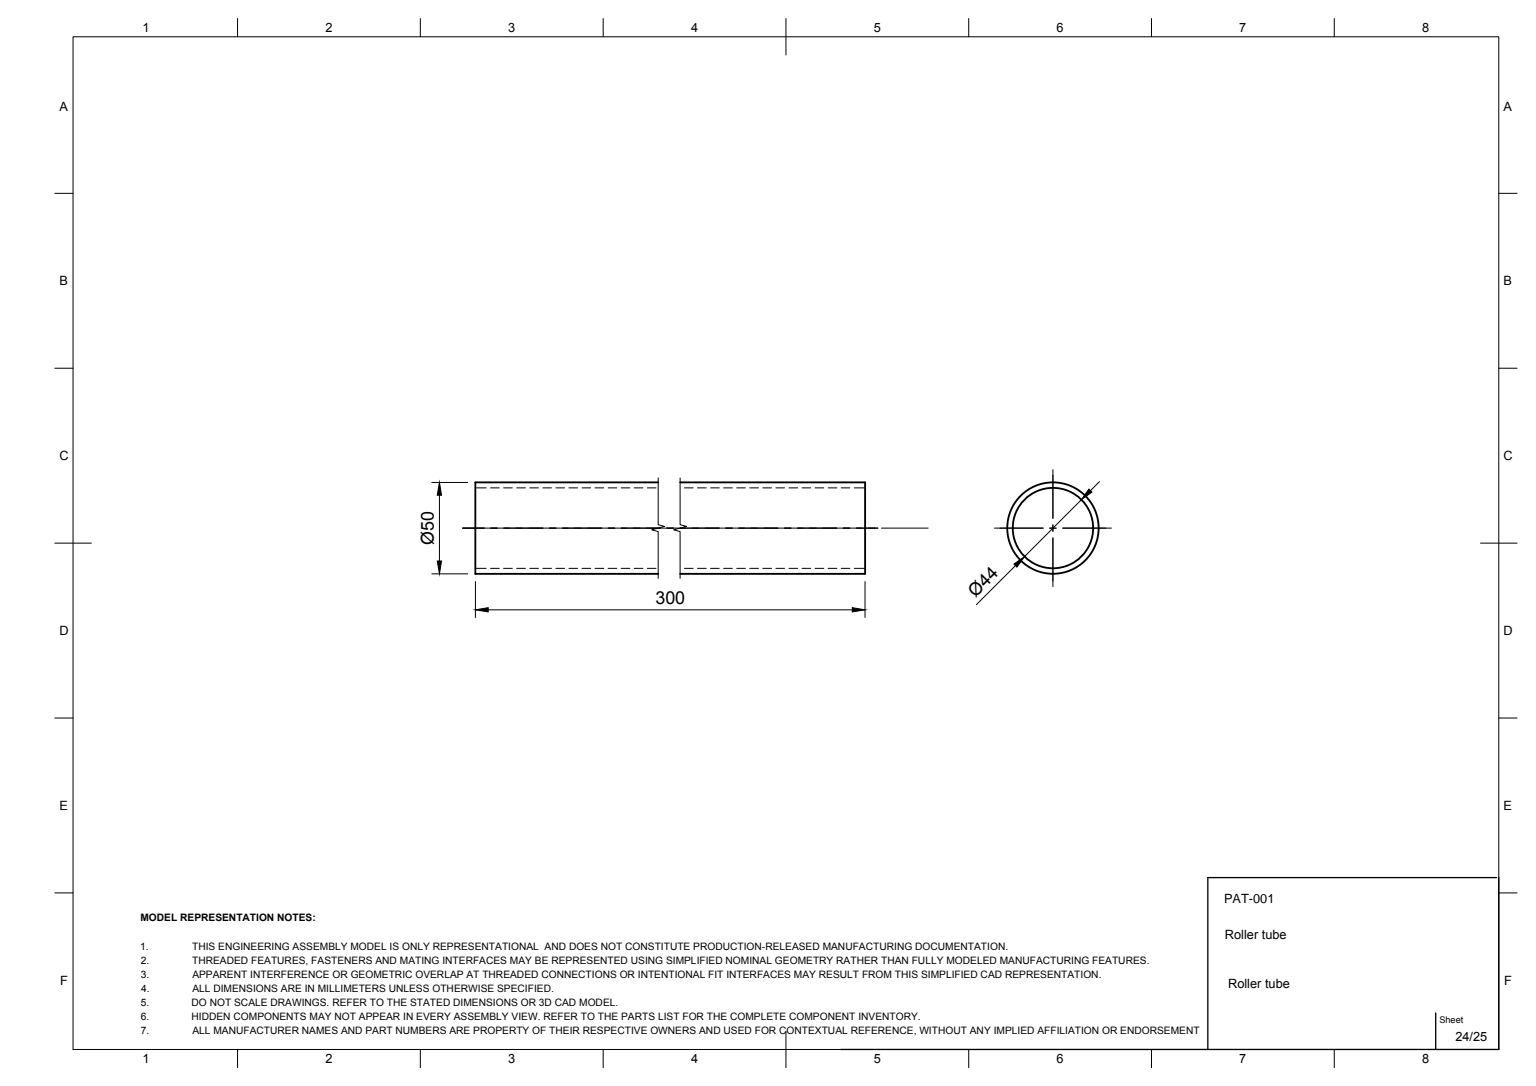
ISO-10303-21;
HEADER;
/* Generated by software containing ST-Developer
 * from STEP Tools, Inc. (www.steptools.com) 
 */

FILE_DESCRIPTION(
/* description */ ('PAT-001'),
/* implementation_level */ '2;1');

FILE_NAME(
/* name */ 'Roller tube.step',
/* time_stamp */ '2026-10-29T17:07:15-07:00',
/* author */ (''),
/* organization */ (''),
/* preprocessor_version */ 'ST-DEVELOPER v20.2',
/* originating_system */ 'Autodesk Translation Framework v15.17.0.0',
/* authorisation */ '');

FILE_SCHEMA (('AUTOMOTIVE_DESIGN { 1 0 10303 214 3 1 1 }'));
ENDSEC;

DATA;
#10=MECHANICAL_DESIGN_GEOMETRIC_PRESENTATION_REPRESENTATION('',(#403),#9622);
#345=SHAPE_REPRESENTATION_RELATIONSHIP('SRR','None',#9770,#370);
#370=ADVANCED_BREP_SHAPE_REPRESENTATION('',(#435),#9619);
#403=STYLED_ITEM('',(#9948),#435);
#435=MANIFOLD_SOLID_BREP('Body1',#5229);
#515=FACE_BOUND('',#1359,.T.);
#516=FACE_BOUND('',#1361,.T.);
#700=PLANE('',#6004);
#701=PLANE('',#6005);
#982=FACE_OUTER_BOUND('',#1356,.T.);
#983=FACE_OUTER_BOUND('',#1357,.T.);
#984=FACE_OUTER_BOUND('',#1358,.T.);
#985=FACE_OUTER_BOUND('',#1360,.T.);
#1356=EDGE_LOOP('',(#4715,#4716,#4717,#4718));
#1357=EDGE_LOOP('',(#4719,#4720,#4721,#4722));
#1358=EDGE_LOOP('',(#4723));
#1359=EDGE_LOOP('',(#4724));
#1360=EDGE_LOOP('',(#4725));
#1361=EDGE_LOOP('',(#4726));
#1771=LINE('',#9390,#2176);
#1772=LINE('',#9396,#2177);
#2176=VECTOR('',#7462,2.2);
#2177=VECTOR('',#7469,2.5);
#2396=CIRCLE('',#5999,2.2);
#2397=CIRCLE('',#6000,2.2);
#2398=CIRCLE('',#6002,2.5);
#2399=CIRCLE('',#6003,2.5);
#2826=VERTEX_POINT('',#9387);
#2827=VERTEX_POINT('',#9389);
#2828=VERTEX_POINT('',#9393);
#2829=VERTEX_POINT('',#9395);
#3461=EDGE_CURVE('',#2826,#2826,#2396,.T.);
#3462=EDGE_CURVE('',#2826,#2827,#1771,.T.);
#3463=EDGE_CURVE('',#2827,#2827,#2397,.T.);
#3464=EDGE_CURVE('',#2828,#2828,#2398,.T.);
#3465=EDGE_CURVE('',#2828,#2829,#1772,.T.);
#3466=EDGE_CURVE('',#2829,#2829,#2399,.T.);
#4715=ORIENTED_EDGE('',*,*,#3461,.F.);
#4716=ORIENTED_EDGE('',*,*,#3462,.T.);
#4717=ORIENTED_EDGE('',*,*,#3463,.T.);
#4718=ORIENTED_EDGE('',*,*,#3462,.F.);
#4719=ORIENTED_EDGE('',*,*,#3464,.F.);
#4720=ORIENTED_EDGE('',*,*,#3465,.T.);
#4721=ORIENTED_EDGE('',*,*,#3466,.T.);
#4722=ORIENTED_EDGE('',*,*,#3465,.F.);
#4723=ORIENTED_EDGE('',*,*,#3464,.T.);
#4724=ORIENTED_EDGE('',*,*,#3461,.T.);
#4725=ORIENTED_EDGE('',*,*,#3466,.F.);
#4726=ORIENTED_EDGE('',*,*,#3463,.F.);
#4892=CYLINDRICAL_SURFACE('',#5998,2.2);
#4893=CYLINDRICAL_SURFACE('',#6001,2.5);
#5169=ADVANCED_FACE('',(#982),#4892,.F.);
#5170=ADVANCED_FACE('',(#983),#4893,.T.);
#5171=ADVANCED_FACE('',(#984,#515),#700,.T.);
#5172=ADVANCED_FACE('',(#985,#516),#701,.F.);
#5229=CLOSED_SHELL('',(#5169,#5170,#5171,#5172));
#5997=AXIS2_PLACEMENT_3D('',#9385,#7456,#7457);
#5998=AXIS2_PLACEMENT_3D('',#9386,#7458,#7459);
#5999=AXIS2_PLACEMENT_3D('',#9388,#7460,#7461);
#6000=AXIS2_PLACEMENT_3D('',#9391,#7463,#7464);
#6001=AXIS2_PLACEMENT_3D('',#9392,#7465,#7466);
#6002=AXIS2_PLACEMENT_3D('',#9394,#7467,#7468);
#6003=AXIS2_PLACEMENT_3D('',#9397,#7470,#7471);
#6004=AXIS2_PLACEMENT_3D('',#9398,#7472,#7473);
#6005=AXIS2_PLACEMENT_3D('',#9399,#7474,#7475);
#7456=DIRECTION('axis',(0.,0.,1.));
#7457=DIRECTION('refdir',(1.,0.,0.));
#7458=DIRECTION('center_axis',(0.,1.,0.));
#7459=DIRECTION('ref_axis',(1.,0.,0.));
#7460=DIRECTION('center_axis',(0.,-1.,0.));
#7461=DIRECTION('ref_axis',(1.,0.,0.));
#7462=DIRECTION('',(0.,-1.,0.));
#7463=DIRECTION('center_axis',(0.,-1.,0.));
#7464=DIRECTION('ref_axis',(1.,0.,0.));
#7465=DIRECTION('center_axis',(0.,1.,0.));
#7466=DIRECTION('ref_axis',(1.,0.,0.));
#7467=DIRECTION('center_axis',(0.,1.,0.));
#7468=DIRECTION('ref_axis',(1.,0.,0.));
#7469=DIRECTION('',(0.,-1.,0.));
#7470=DIRECTION('center_axis',(0.,1.,0.));
#7471=DIRECTION('ref_axis',(1.,0.,0.));
#7472=DIRECTION('center_axis',(0.,1.,0.));
#7473=DIRECTION('ref_axis',(1.,0.,0.));
#7474=DIRECTION('center_axis',(0.,1.,0.));
#7475=DIRECTION('ref_axis',(1.,0.,0.));
#9385=CARTESIAN_POINT('',(0.,0.,0.));
#9386=CARTESIAN_POINT('Origin',(0.,0.,4.5));
#9387=CARTESIAN_POINT('',(-2.2,30.,4.5));
#9388=CARTESIAN_POINT('Origin',(0.,30.,4.5));
#9389=CARTESIAN_POINT('',(-2.2,0.,4.5));
#9390=CARTESIAN_POINT('',(-2.2,0.,4.5));
#9391=CARTESIAN_POINT('Origin',(0.,0.,4.5));
#9392=CARTESIAN_POINT('Origin',(0.,0.,4.5));
#9393=CARTESIAN_POINT('',(-2.5,30.,4.5));
#9394=CARTESIAN_POINT('Origin',(0.,30.,4.5));
#9395=CARTESIAN_POINT('',(-2.5,0.,4.5));
#9396=CARTESIAN_POINT('',(-2.5,0.,4.5));
#9397=CARTESIAN_POINT('Origin',(0.,0.,4.5));
#9398=CARTESIAN_POINT('Origin',(0.,30.,4.5));
#9399=CARTESIAN_POINT('Origin',(0.,0.,4.5));
#9589=UNCERTAINTY_MEASURE_WITH_UNIT(LENGTH_MEASURE(0.001),#9623,
'DISTANCE_ACCURACY_VALUE',
'Maximum model space distance between geometric entities at asserted c
onnectivities');
#9592=UNCERTAINTY_MEASURE_WITH_UNIT(LENGTH_MEASURE(0.001),#9623,
'DISTANCE_ACCURACY_VALUE',
'Maximum model space distance between geometric entities at asserted c
onnectivities');
#9619=(
GEOMETRIC_REPRESENTATION_CONTEXT(3)
GLOBAL_UNCERTAINTY_ASSIGNED_CONTEXT((#9589))
GLOBAL_UNIT_ASSIGNED_CONTEXT((#9623,#9625,#9626))
REPRESENTATION_CONTEXT('','3D')
);
#9622=(
GEOMETRIC_REPRESENTATION_CONTEXT(3)
GLOBAL_UNCERTAINTY_ASSIGNED_CONTEXT((#9592))
GLOBAL_UNIT_ASSIGNED_CONTEXT((#9623,#9625,#9626))
REPRESENTATION_CONTEXT('','3D')
);
#9623=(
LENGTH_UNIT()
NAMED_UNIT(*)
SI_UNIT(.CENTI.,.METRE.)
);
#9625=(
NAMED_UNIT(*)
PLANE_ANGLE_UNIT()
SI_UNIT($,.RADIAN.)
);
#9626=(
NAMED_UNIT(*)
SI_UNIT($,.STERADIAN.)
SOLID_ANGLE_UNIT()
);
#9653=SHAPE_DEFINITION_REPRESENTATION(#9687,#9770);
#9687=PRODUCT_DEFINITION_SHAPE('',$,#9800);
#9770=SHAPE_REPRESENTATION('',(#5997),#9619);
#9773=PRODUCT_DEFINITION_CONTEXT('part definition',#9862,'design');
#9800=PRODUCT_DEFINITION('Roller tube','Roller tube',#9829,#9773);
#9829=PRODUCT_DEFINITION_FORMATION('',$,#9890);
#9862=APPLICATION_CONTEXT(
'Core Data for Automotive Mechanical Design Process');
#9863=PRODUCT_CONTEXT('part definition',#9862,'mechanical');
#9890=PRODUCT('Roller tube','Roller tube','Roller tube',(#9863));
#9942=COLOUR_RGB('Light Blue',0.38,0.62,0.78);
#9943=FILL_AREA_STYLE_COLOUR('',#9942);
#9944=FILL_AREA_STYLE('',(#9943));
#9945=SURFACE_STYLE_FILL_AREA(#9944);
#9946=SURFACE_SIDE_STYLE('',(#9945));
#9947=SURFACE_STYLE_USAGE(.BOTH.,#9946);
#9948=PRESENTATION_STYLE_ASSIGNMENT((#9947));
ENDSEC;
END-ISO-10303-21;
